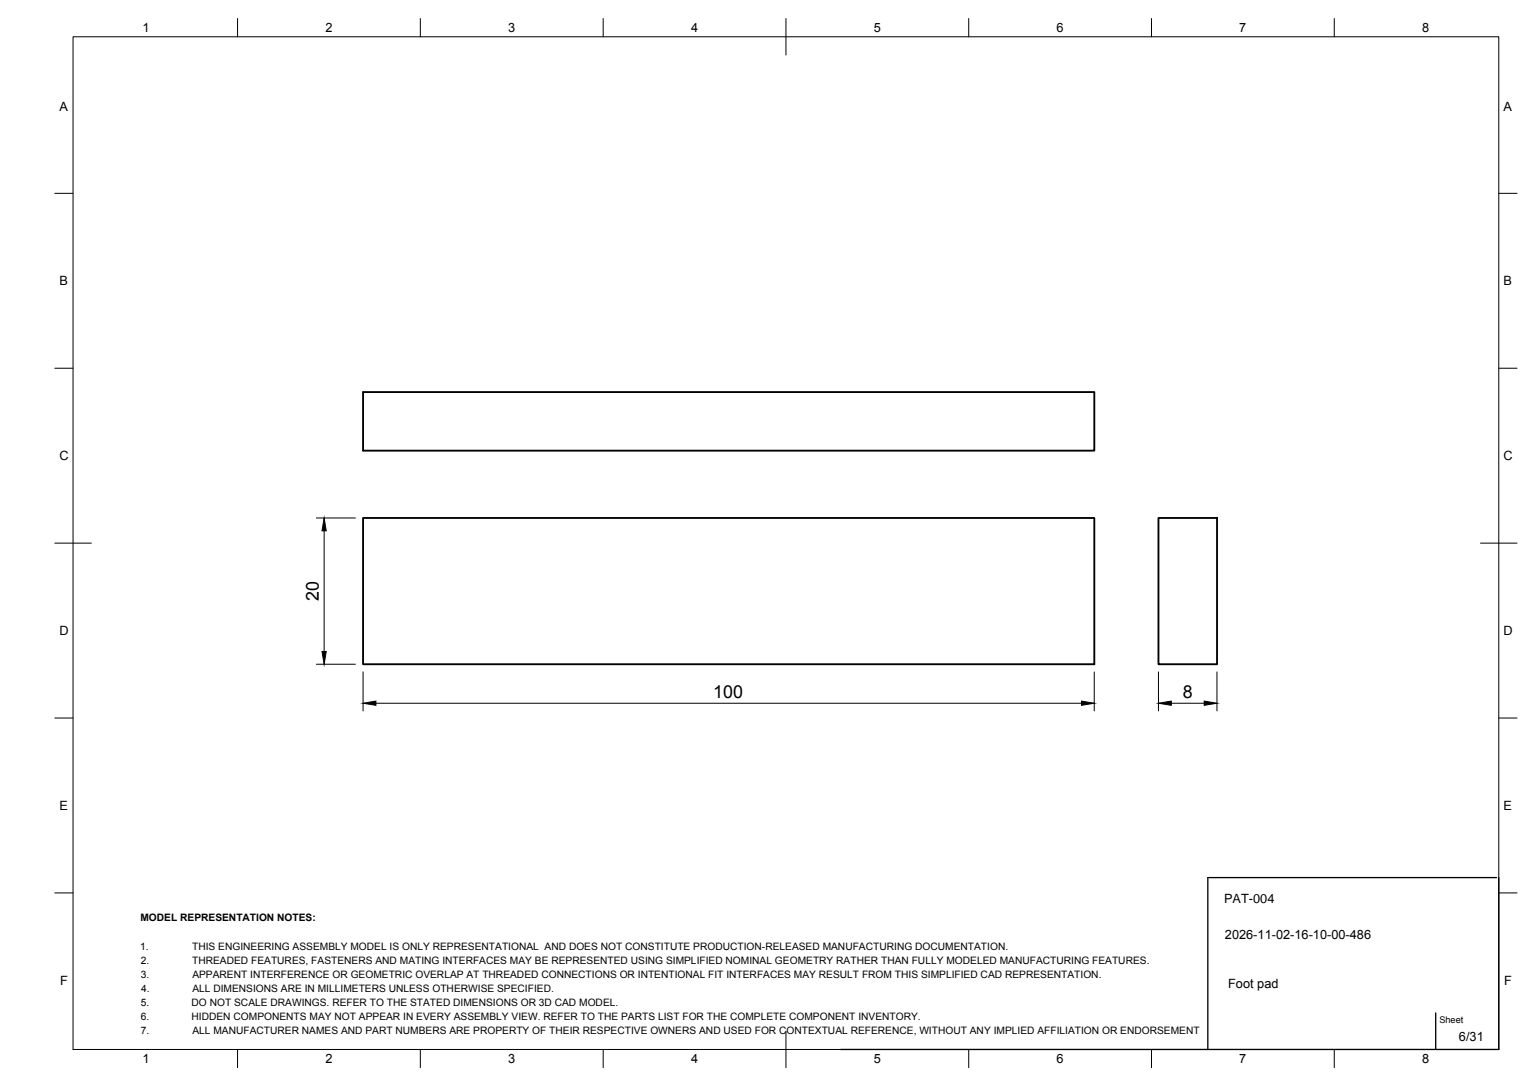
ISO-10303-21;
HEADER;
/* Generated by software containing ST-Developer
 * from STEP Tools, Inc. (www.steptools.com) 
 */

FILE_DESCRIPTION(
/* description */ ('Air blow-off nozzle station'),
/* implementation_level */ '2;1');

FILE_NAME(
/* name */ 'Foot pad.step',
/* time_stamp */ '2026-10-27T10:53:54-07:00',
/* author */ (''),
/* organization */ (''),
/* preprocessor_version */ 'ST-DEVELOPER v20.2',
/* originating_system */ 'Autodesk Translation Framework v15.17.0.0',
/* authorisation */ '');

FILE_SCHEMA (('AUTOMOTIVE_DESIGN { 1 0 10303 214 3 1 1 }'));
ENDSEC;

DATA;
#10=MECHANICAL_DESIGN_GEOMETRIC_PRESENTATION_REPRESENTATION('',(#238),#7897);
#188=SHAPE_REPRESENTATION_RELATIONSHIP('SRR','None',#8002,#213);
#213=ADVANCED_BREP_SHAPE_REPRESENTATION('',(#263),#7869);
#238=STYLED_ITEM('',(#8213),#263);
#263=MANIFOLD_SOLID_BREP('Body1',#4287);
#377=PLANE('',#4602);
#378=PLANE('',#4603);
#379=PLANE('',#4604);
#380=PLANE('',#4605);
#381=PLANE('',#4606);
#382=PLANE('',#4607);
#547=FACE_OUTER_BOUND('',#805,.T.);
#548=FACE_OUTER_BOUND('',#806,.T.);
#549=FACE_OUTER_BOUND('',#807,.T.);
#550=FACE_OUTER_BOUND('',#808,.T.);
#551=FACE_OUTER_BOUND('',#809,.T.);
#552=FACE_OUTER_BOUND('',#810,.T.);
#805=EDGE_LOOP('',(#2927,#2928,#2929,#2930));
#806=EDGE_LOOP('',(#2931,#2932,#2933,#2934));
#807=EDGE_LOOP('',(#2935,#2936,#2937,#2938));
#808=EDGE_LOOP('',(#2939,#2940,#2941,#2942));
#809=EDGE_LOOP('',(#2943,#2944,#2945,#2946));
#810=EDGE_LOOP('',(#2947,#2948,#2949,#2950));
#1151=LINE('',#6431,#1505);
#1152=LINE('',#6433,#1506);
#1153=LINE('',#6435,#1507);
#1154=LINE('',#6436,#1508);
#1155=LINE('',#6439,#1509);
#1156=LINE('',#6441,#1510);
#1157=LINE('',#6442,#1511);
#1158=LINE('',#6445,#1512);
#1159=LINE('',#6447,#1513);
#1160=LINE('',#6448,#1514);
#1161=LINE('',#6450,#1515);
#1162=LINE('',#6451,#1516);
#1505=VECTOR('',#5113,1.);
#1506=VECTOR('',#5114,1.);
#1507=VECTOR('',#5115,1.);
#1508=VECTOR('',#5116,1.);
#1509=VECTOR('',#5119,1.);
#1510=VECTOR('',#5120,1.);
#1511=VECTOR('',#5121,1.);
#1512=VECTOR('',#5124,1.);
#1513=VECTOR('',#5125,1.);
#1514=VECTOR('',#5126,1.);
#1515=VECTOR('',#5129,1.);
#1516=VECTOR('',#5130,1.);
#2017=VERTEX_POINT('',#6429);
#2018=VERTEX_POINT('',#6430);
#2019=VERTEX_POINT('',#6432);
#2020=VERTEX_POINT('',#6434);
#2021=VERTEX_POINT('',#6438);
#2022=VERTEX_POINT('',#6440);
#2023=VERTEX_POINT('',#6444);
#2024=VERTEX_POINT('',#6446);
#2381=EDGE_CURVE('',#2017,#2018,#1151,.T.);
#2382=EDGE_CURVE('',#2018,#2019,#1152,.T.);
#2383=EDGE_CURVE('',#2020,#2019,#1153,.T.);
#2384=EDGE_CURVE('',#2017,#2020,#1154,.T.);
#2385=EDGE_CURVE('',#2021,#2017,#1155,.T.);
#2386=EDGE_CURVE('',#2022,#2020,#1156,.T.);
#2387=EDGE_CURVE('',#2021,#2022,#1157,.T.);
#2388=EDGE_CURVE('',#2023,#2021,#1158,.T.);
#2389=EDGE_CURVE('',#2024,#2022,#1159,.T.);
#2390=EDGE_CURVE('',#2023,#2024,#1160,.T.);
#2391=EDGE_CURVE('',#2018,#2023,#1161,.T.);
#2392=EDGE_CURVE('',#2019,#2024,#1162,.T.);
#2927=ORIENTED_EDGE('',*,*,#2381,.T.);
#2928=ORIENTED_EDGE('',*,*,#2382,.T.);
#2929=ORIENTED_EDGE('',*,*,#2383,.F.);
#2930=ORIENTED_EDGE('',*,*,#2384,.F.);
#2931=ORIENTED_EDGE('',*,*,#2385,.T.);
#2932=ORIENTED_EDGE('',*,*,#2384,.T.);
#2933=ORIENTED_EDGE('',*,*,#2386,.F.);
#2934=ORIENTED_EDGE('',*,*,#2387,.F.);
#2935=ORIENTED_EDGE('',*,*,#2388,.T.);
#2936=ORIENTED_EDGE('',*,*,#2387,.T.);
#2937=ORIENTED_EDGE('',*,*,#2389,.F.);
#2938=ORIENTED_EDGE('',*,*,#2390,.F.);
#2939=ORIENTED_EDGE('',*,*,#2391,.T.);
#2940=ORIENTED_EDGE('',*,*,#2390,.T.);
#2941=ORIENTED_EDGE('',*,*,#2392,.F.);
#2942=ORIENTED_EDGE('',*,*,#2382,.F.);
#2943=ORIENTED_EDGE('',*,*,#2392,.T.);
#2944=ORIENTED_EDGE('',*,*,#2389,.T.);
#2945=ORIENTED_EDGE('',*,*,#2386,.T.);
#2946=ORIENTED_EDGE('',*,*,#2383,.T.);
#2947=ORIENTED_EDGE('',*,*,#2391,.F.);
#2948=ORIENTED_EDGE('',*,*,#2381,.F.);
#2949=ORIENTED_EDGE('',*,*,#2385,.F.);
#2950=ORIENTED_EDGE('',*,*,#2388,.F.);
#4037=ADVANCED_FACE('',(#547),#377,.T.);
#4038=ADVANCED_FACE('',(#548),#378,.T.);
#4039=ADVANCED_FACE('',(#549),#379,.T.);
#4040=ADVANCED_FACE('',(#550),#380,.T.);
#4041=ADVANCED_FACE('',(#551),#381,.T.);
#4042=ADVANCED_FACE('',(#552),#382,.F.);
#4287=CLOSED_SHELL('',(#4037,#4038,#4039,#4040,#4041,#4042));
#4601=AXIS2_PLACEMENT_3D('',#6427,#5109,#5110);
#4602=AXIS2_PLACEMENT_3D('',#6428,#5111,#5112);
#4603=AXIS2_PLACEMENT_3D('',#6437,#5117,#5118);
#4604=AXIS2_PLACEMENT_3D('',#6443,#5122,#5123);
#4605=AXIS2_PLACEMENT_3D('',#6449,#5127,#5128);
#4606=AXIS2_PLACEMENT_3D('',#6452,#5131,#5132);
#4607=AXIS2_PLACEMENT_3D('',#6453,#5133,#5134);
#5109=DIRECTION('axis',(0.,0.,1.));
#5110=DIRECTION('refdir',(1.,0.,0.));
#5111=DIRECTION('center_axis',(0.,1.,0.));
#5112=DIRECTION('ref_axis',(-1.,0.,0.));
#5113=DIRECTION('',(-1.,0.,0.));
#5114=DIRECTION('',(0.,0.,1.));
#5115=DIRECTION('',(-1.,0.,0.));
#5116=DIRECTION('',(0.,0.,1.));
#5117=DIRECTION('center_axis',(1.,0.,0.));
#5118=DIRECTION('ref_axis',(0.,1.,0.));
#5119=DIRECTION('',(0.,1.,0.));
#5120=DIRECTION('',(0.,1.,0.));
#5121=DIRECTION('',(0.,0.,1.));
#5122=DIRECTION('center_axis',(0.,-1.,0.));
#5123=DIRECTION('ref_axis',(1.,0.,0.));
#5124=DIRECTION('',(1.,0.,0.));
#5125=DIRECTION('',(1.,0.,0.));
#5126=DIRECTION('',(0.,0.,1.));
#5127=DIRECTION('center_axis',(-1.,0.,0.));
#5128=DIRECTION('ref_axis',(0.,-1.,0.));
#5129=DIRECTION('',(0.,-1.,0.));
#5130=DIRECTION('',(0.,-1.,0.));
#5131=DIRECTION('center_axis',(0.,0.,1.));
#5132=DIRECTION('ref_axis',(1.,0.,0.));
#5133=DIRECTION('center_axis',(0.,0.,1.));
#5134=DIRECTION('ref_axis',(1.,0.,0.));
#6427=CARTESIAN_POINT('',(0.,0.,0.));
#6428=CARTESIAN_POINT('Origin',(-4.,6.,-0.8));
#6429=CARTESIAN_POINT('',(-4.,6.,-0.8));
#6430=CARTESIAN_POINT('',(-6.,6.,-0.8));
#6431=CARTESIAN_POINT('',(-4.,6.,-0.8));
#6432=CARTESIAN_POINT('',(-6.,6.,0.));
#6433=CARTESIAN_POINT('',(-6.,6.,-0.8));
#6434=CARTESIAN_POINT('',(-4.,6.,0.));
#6435=CARTESIAN_POINT('',(-4.,6.,0.));
#6436=CARTESIAN_POINT('',(-4.,6.,-0.8));
#6437=CARTESIAN_POINT('Origin',(-4.,-4.,-0.8));
#6438=CARTESIAN_POINT('',(-4.,-4.,-0.8));
#6439=CARTESIAN_POINT('',(-4.,-4.,-0.8));
#6440=CARTESIAN_POINT('',(-4.,-4.,0.));
#6441=CARTESIAN_POINT('',(-4.,-4.,0.));
#6442=CARTESIAN_POINT('',(-4.,-4.,-0.8));
#6443=CARTESIAN_POINT('Origin',(-6.,-4.,-0.8));
#6444=CARTESIAN_POINT('',(-6.,-4.,-0.8));
#6445=CARTESIAN_POINT('',(-6.,-4.,-0.8));
#6446=CARTESIAN_POINT('',(-6.,-4.,0.));
#6447=CARTESIAN_POINT('',(-6.,-4.,0.));
#6448=CARTESIAN_POINT('',(-6.,-4.,-0.8));
#6449=CARTESIAN_POINT('Origin',(-6.,6.,-0.8));
#6450=CARTESIAN_POINT('',(-6.,6.,-0.8));
#6451=CARTESIAN_POINT('',(-6.,6.,0.));
#6452=CARTESIAN_POINT('Origin',(-5.,1.,0.));
#6453=CARTESIAN_POINT('Origin',(-5.,1.,-0.8));
#7837=UNCERTAINTY_MEASURE_WITH_UNIT(LENGTH_MEASURE(0.001),#7898,
'DISTANCE_ACCURACY_VALUE',
'Maximum model space distance between geometric entities at asserted c
onnectivities');
#7865=UNCERTAINTY_MEASURE_WITH_UNIT(LENGTH_MEASURE(0.001),#7898,
'DISTANCE_ACCURACY_VALUE',
'Maximum model space distance between geometric entities at asserted c
onnectivities');
#7869=(
GEOMETRIC_REPRESENTATION_CONTEXT(3)
GLOBAL_UNCERTAINTY_ASSIGNED_CONTEXT((#7837))
GLOBAL_UNIT_ASSIGNED_CONTEXT((#7898,#7900,#7901))
REPRESENTATION_CONTEXT('','3D')
);
#7897=(
GEOMETRIC_REPRESENTATION_CONTEXT(3)
GLOBAL_UNCERTAINTY_ASSIGNED_CONTEXT((#7865))
GLOBAL_UNIT_ASSIGNED_CONTEXT((#7898,#7900,#7901))
REPRESENTATION_CONTEXT('','3D')
);
#7898=(
LENGTH_UNIT()
NAMED_UNIT(*)
SI_UNIT(.CENTI.,.METRE.)
);
#7900=(
NAMED_UNIT(*)
PLANE_ANGLE_UNIT()
SI_UNIT($,.RADIAN.)
);
#7901=(
NAMED_UNIT(*)
SI_UNIT($,.STERADIAN.)
SOLID_ANGLE_UNIT()
);
#7905=SHAPE_DEFINITION_REPRESENTATION(#7936,#8002);
#7936=PRODUCT_DEFINITION_SHAPE('',$,#8034);
#8002=SHAPE_REPRESENTATION('',(#4601),#7869);
#8030=PRODUCT_DEFINITION_CONTEXT('part definition',#8125,'design');
#8034=PRODUCT_DEFINITION('Foot pad','Foot pad',#8065,#8030);
#8065=PRODUCT_DEFINITION_FORMATION('',$,#8130);
#8125=APPLICATION_CONTEXT(
'Core Data for Automotive Mechanical Design Process');
#8126=PRODUCT_CONTEXT('part definition',#8125,'mechanical');
#8130=PRODUCT('Foot pad','Foot pad','Foot pad',(#8126));
#8207=COLOUR_RGB('Sky Blue',0.24,0.69,0.87);
#8208=FILL_AREA_STYLE_COLOUR('',#8207);
#8209=FILL_AREA_STYLE('',(#8208));
#8210=SURFACE_STYLE_FILL_AREA(#8209);
#8211=SURFACE_SIDE_STYLE('',(#8210));
#8212=SURFACE_STYLE_USAGE(.BOTH.,#8211);
#8213=PRESENTATION_STYLE_ASSIGNMENT((#8212));
ENDSEC;
END-ISO-10303-21;
